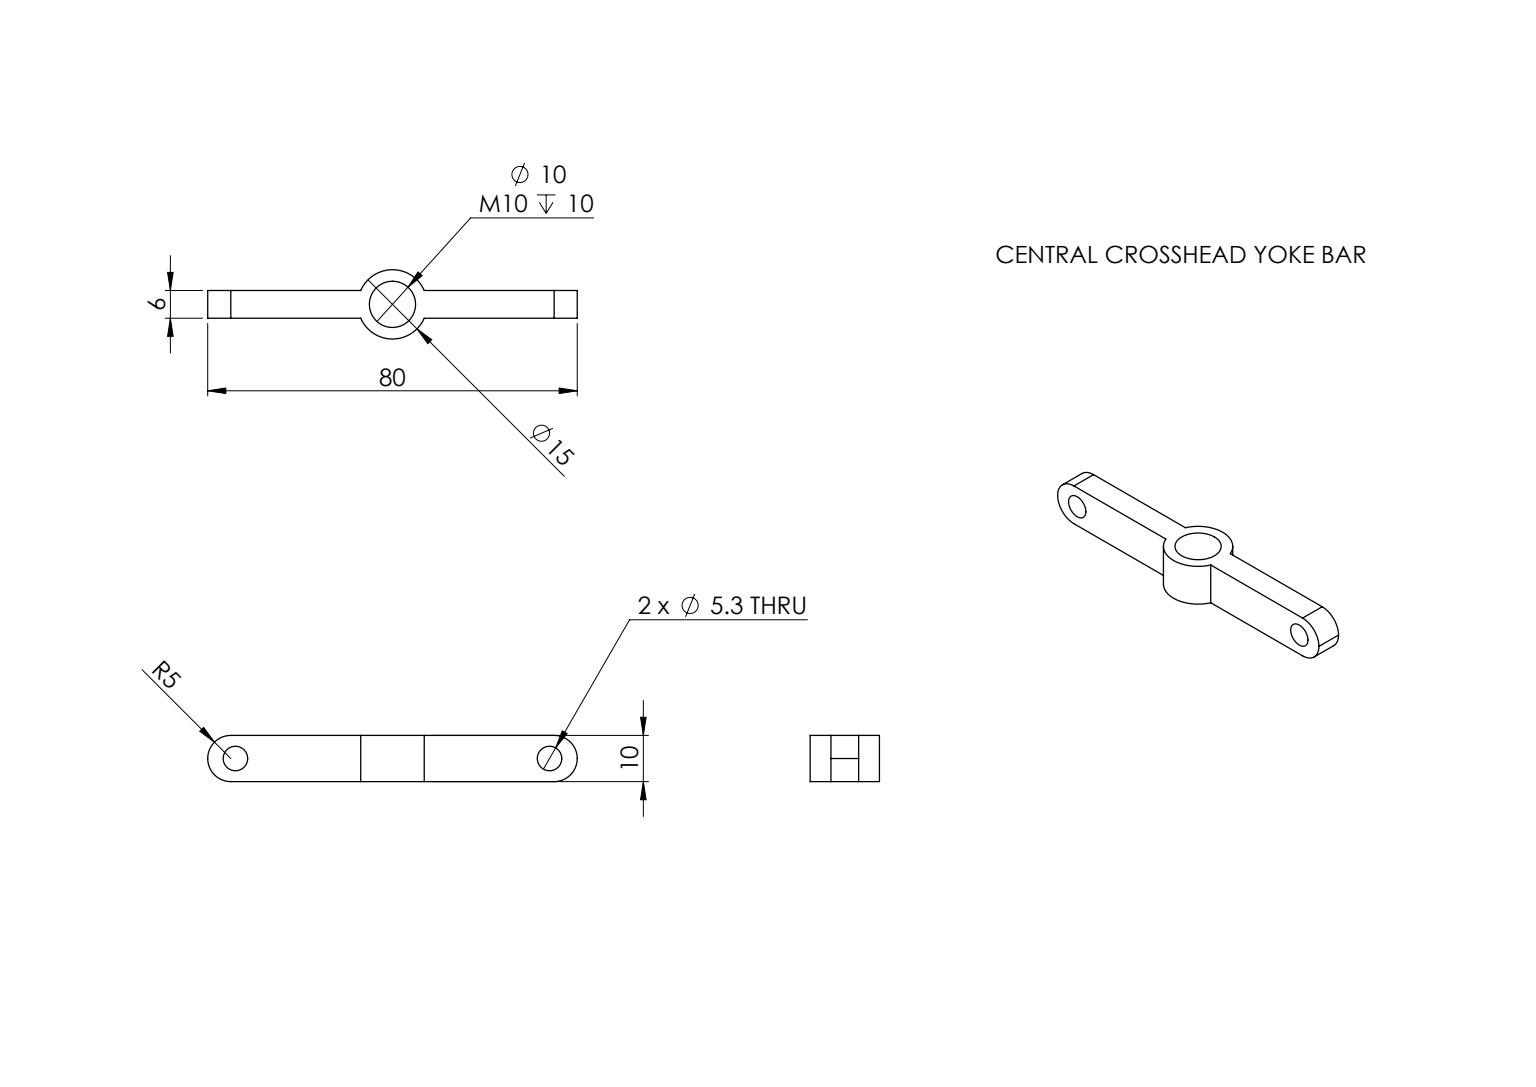
ISO-10303-21;
HEADER;
FILE_DESCRIPTION (('STEP AP214'),
    '1' );
FILE_NAME ('Central Crosshead Yoke Bar.step',
    '2026-10-22T13:24:12',
    ( '' ),
    ( '' ),
    'SwSTEP 2.0',
    'SolidWorks 2026',
    '' );
FILE_SCHEMA (( 'AUTOMOTIVE_DESIGN' ));
ENDSEC;

DATA;
#8=ORIENTED_EDGE ( 'NONE', *, *, #1854, .F. ) ;
#23=VERTEX_POINT ( 'NONE', #2540 ) ;
#29=ORIENTED_EDGE ( 'NONE', *, *, #1848, .F. ) ;
#30=DIRECTION ( 'NONE',  ( -1.000000000000000000, 0.000000000000000000, 0.000000000000000000 ) ) ;
#34=ORIENTED_EDGE ( 'NONE', *, *, #947, .F. ) ;
#40=SURFACE_SIDE_STYLE ('',( #2060 ) ) ;
#41=ORIENTED_EDGE ( 'NONE', *, *, #2625, .F. ) ;
#43=DIRECTION ( 'NONE',  ( -0.000000000000000000, -1.000000000000000000, -0.000000000000000000 ) ) ;
#44=DIRECTION ( 'NONE',  ( 0.000000000000000000, 1.000000000000000000, 0.000000000000000000 ) ) ;
#48=CARTESIAN_POINT ( 'NONE',  ( -34.99999999999999289, -20.00000000000000000, 3.000000000000000000 ) ) ;
#49=CIRCLE ( 'NONE', #831, 7.500000000000000888 ) ;
#50=FACE_BOUND ( 'NONE', #2831, .T. ) ;
#61=DIRECTION ( 'NONE',  ( 1.000000000000000000, 0.000000000000000000, 0.000000000000000000 ) ) ;
#64=ORIENTED_EDGE ( 'NONE', *, *, #1925, .F. ) ;
#65=EDGE_CURVE ( 'NONE', #415, #110, #2593, .T. ) ;
#67=AXIS2_PLACEMENT_3D ( 'NONE', #278, #535, #1657 ) ;
#80=EDGE_CURVE ( 'NONE', #1900, #237, #994, .T. ) ;
#84=CARTESIAN_POINT ( 'NONE',  ( -39.99999999999999289, -30.00000000000000000, -3.000000000000000000 ) ) ;
#97=STYLED_ITEM('',(#2949),#2534);
#99=CARTESIAN_POINT ( 'NONE',  ( -31.35000000000001563, -25.00000000000000000, -3.000000000000001332 ) ) ;
#100=EDGE_LOOP ( 'NONE', ( #2045, #2281 ) ) ;
#101=MECHANICAL_DESIGN_GEOMETRIC_PRESENTATION_REPRESENTATION('',(#833),#2032);
#102=DIRECTION ( 'NONE',  ( -1.000000000000000000, 0.000000000000000000, 0.000000000000000000 ) ) ;
#110=VERTEX_POINT ( 'NONE', #332 ) ;
#112=VECTOR ( 'NONE', #2880, 1000.000000000000000 ) ;
#115=EDGE_LOOP ( 'NONE', ( #29, #1418, #842, #2140 ) ) ;
#130=ORIENTED_EDGE ( 'NONE', *, *, #1665, .T. ) ;
#133=DIRECTION ( 'NONE',  ( -2.312964634635742661E-15, 0.000000000000000000, -1.000000000000000000 ) ) ;
#135=ORIENTED_EDGE ( 'NONE', *, *, #1188, .F. ) ;
#144=DIRECTION ( 'NONE',  ( 1.000000000000000000, 0.000000000000000000, -2.341876692568690761E-15 ) ) ;
#147=CYLINDRICAL_SURFACE ( 'NONE', #663, 5.000000000000000888 ) ;
#157=EDGE_LOOP ( 'NONE', ( #1667, #2865, #926, #590, #162 ) ) ;
#158=VECTOR ( 'NONE', #1568, 1000.000000000000000 ) ;
#162=ORIENTED_EDGE ( 'NONE', *, *, #1048, .T. ) ;
#163=FACE_OUTER_BOUND ( 'NONE', #394, .T. ) ;
#165=EDGE_LOOP ( 'NONE', ( #896, #1637 ) ) ;
#166=( NAMED_UNIT ( * ) SI_UNIT ( $, .STERADIAN. ) SOLID_ANGLE_UNIT ( ) );
#170=CARTESIAN_POINT ( 'NONE',  ( 34.00000000000000000, -25.00000000000000000, -3.000000000000001332 ) ) ;
#174=ORIENTED_EDGE ( 'NONE', *, *, #892, .F. ) ;
#179=CARTESIAN_POINT ( 'NONE',  ( -6.873863542433761076, -20.00000000000000000, 3.000000000000000000 ) ) ;
#187=DIRECTION ( 'NONE',  ( -0.000000000000000000, -1.000000000000000000, -0.000000000000000000 ) ) ;
#193=AXIS2_PLACEMENT_3D ( 'NONE', #1698, #1267, #144 ) ;
#200=FACE_OUTER_BOUND ( 'NONE', #1652, .T. ) ;
#203=ORIENTED_EDGE ( 'NONE', *, *, #1188, .T. ) ;
#206=AXIS2_PLACEMENT_3D ( 'NONE', #1277, #1543, #609 ) ;
#209=DIRECTION ( 'NONE',  ( 0.000000000000000000, 0.000000000000000000, 1.000000000000000000 ) ) ;
#218=VERTEX_POINT ( 'NONE', #1654 ) ;
#220=PLANE ( 'NONE',  #1032 ) ;
#221=DIRECTION ( 'NONE',  ( 0.000000000000000000, 0.000000000000000000, -1.000000000000000000 ) ) ;
#227=CARTESIAN_POINT ( 'NONE',  ( 0.000000000000000000, -30.00000000000000000, 0.000000000000000000 ) ) ;
#228=DIRECTION ( 'NONE',  ( -0.000000000000000000, -1.000000000000000000, -0.000000000000000000 ) ) ;
#231=CARTESIAN_POINT ( 'NONE',  ( 0.000000000000000000, 0.000000000000000000, 0.000000000000000000 ) ) ;
#237=VERTEX_POINT ( 'NONE', #1323 ) ;
#239=AXIS2_PLACEMENT_3D ( 'NONE', #267, #1061, #1149 ) ;
#241=ORIENTED_EDGE ( 'NONE', *, *, #2815, .T. ) ;
#244=ADVANCED_FACE ( 'NONE', ( #397 ), #1289, .T. ) ;
#246=EDGE_CURVE ( 'NONE', #218, #2864, #2203, .T. ) ;
#256=VECTOR ( 'NONE', #2846, 1000.000000000000000 ) ;
#258=EDGE_LOOP ( 'NONE', ( #2402, #1202, #483, #1037 ) ) ;
#259=LINE ( 'NONE', #2309, #1324 ) ;
#264=EDGE_LOOP ( 'NONE', ( #1087, #283, #1551, #1453 ) ) ;
#267=CARTESIAN_POINT ( 'NONE',  ( -34.00000000000000000, -25.00000000000000000, -3.000000000000000000 ) ) ;
#271=ADVANCED_FACE ( 'NONE', ( #1528 ), #592, .T. ) ;
#275=ORIENTED_EDGE ( 'NONE', *, *, #574, .T. ) ;
#276=DIRECTION ( 'NONE',  ( -1.000000000000000000, 0.000000000000000000, 0.000000000000000000 ) ) ;
#278=CARTESIAN_POINT ( 'NONE',  ( 34.00000000000000000, -25.00000000000000000, -3.000000000000001332 ) ) ;
#283=ORIENTED_EDGE ( 'NONE', *, *, #2016, .F. ) ;
#284=DIRECTION ( 'NONE',  ( 0.000000000000000000, -0.000000000000000000, 1.000000000000000000 ) ) ;
#285=( GEOMETRIC_REPRESENTATION_CONTEXT ( 3 ) GLOBAL_UNCERTAINTY_ASSIGNED_CONTEXT ( ( #2051 ) ) GLOBAL_UNIT_ASSIGNED_CONTEXT ( ( #2879, #1600, #166 ) ) REPRESENTATION_CONTEXT ( 'NONE', 'WORKASPACE' ) );
#292=LINE ( 'NONE', #1175, #703 ) ;
#293=EDGE_CURVE ( 'NONE', #444, #937, #848, .T. ) ;
#297=CARTESIAN_POINT ( 'NONE',  ( 36.64999999999999147, -25.00000000000000000, -3.000000000000001332 ) ) ;
#299=AXIS2_PLACEMENT_3D ( 'NONE', #2890, #509, #2101 ) ;
#304=ORIENTED_EDGE ( 'NONE', *, *, #2625, .T. ) ;
#313=CARTESIAN_POINT ( 'NONE',  ( 0.000000000000000000, -30.00000000000000000, 0.000000000000000000 ) ) ;
#314=ORIENTED_EDGE ( 'NONE', *, *, #2815, .F. ) ;
#318=ADVANCED_FACE ( 'NONE', ( #200 ), #1081, .F. ) ;
#320=ORIENTED_EDGE ( 'NONE', *, *, #2703, .T. ) ;
#323=DIRECTION ( 'NONE',  ( 0.000000000000000000, 1.000000000000000000, 0.000000000000000000 ) ) ;
#327=VERTEX_POINT ( 'NONE', #425 ) ;
#328=CIRCLE ( 'NONE', #2312, 7.500000000000000888 ) ;
#331=CIRCLE ( 'NONE', #981, 5.000000000000000888 ) ;
#332=CARTESIAN_POINT ( 'NONE',  ( 6.873863542433761076, -30.00000000000000000, 3.000000000000000000 ) ) ;
#335=CARTESIAN_POINT ( 'NONE',  ( -34.00000000000000000, -25.00000000000000000, -3.000000000000001332 ) ) ;
#343=AXIS2_PLACEMENT_3D ( 'NONE', #865, #2176, #2444 ) ;
#345=CARTESIAN_POINT ( 'NONE',  ( 6.873863542433761076, -30.00000000000000000, 3.000000000000000000 ) ) ;
#348=VECTOR ( 'NONE', #1776, 1000.000000000000000 ) ;
#354=CARTESIAN_POINT ( 'NONE',  ( 0.000000000000000000, -30.00000000000000000, 0.000000000000000000 ) ) ;
#362=CARTESIAN_POINT ( 'NONE',  ( -34.00000000000000000, -25.00000000000000000, -3.000000000000001332 ) ) ;
#367=DIRECTION ( 'NONE',  ( -0.000000000000000000, -0.000000000000000000, -1.000000000000000000 ) ) ;
#368=ORIENTED_EDGE ( 'NONE', *, *, #2549, .T. ) ;
#370=ADVANCED_FACE ( 'NONE', ( #2055, #484 ), #680, .T. ) ;
#377=CIRCLE ( 'NONE', #602, 7.500000000000000888 ) ;
#383=CIRCLE ( 'NONE', #2037, 2.649999999999992806 ) ;
#393=DIRECTION ( 'NONE',  ( -0.000000000000000000, -0.000000000000000000, -1.000000000000000000 ) ) ;
#394=EDGE_LOOP ( 'NONE', ( #2893, #2844, #823, #135 ) ) ;
#395=CYLINDRICAL_SURFACE ( 'NONE', #239, 2.649999999999992806 ) ;
#397=FACE_OUTER_BOUND ( 'NONE', #2041, .T. ) ;
#403=CARTESIAN_POINT ( 'NONE',  ( -31.35000000000000853, -25.00000000000000000, -3.000000000000000000 ) ) ;
#407=ORIENTED_EDGE ( 'NONE', *, *, #246, .F. ) ;
#411=ORIENTED_EDGE ( 'NONE', *, *, #1925, .T. ) ;
#415=VERTEX_POINT ( 'NONE', #2763 ) ;
#425=CARTESIAN_POINT ( 'NONE',  ( 40.00000000000002132, -24.99999999999999645, 3.000000000000000000 ) ) ;
#426=ADVANCED_FACE ( 'NONE', ( #1140 ), #715, .F. ) ;
#429=ORIENTED_EDGE ( 'NONE', *, *, #1791, .T. ) ;
#442=ORIENTED_EDGE ( 'NONE', *, *, #787, .T. ) ;
#443=CARTESIAN_POINT ( 'NONE',  ( -34.99999999999999289, -30.00000000000000000, -3.000000000000000000 ) ) ;
#444=VERTEX_POINT ( 'NONE', #48 ) ;
#448=LINE ( 'NONE', #1584, #348 ) ;
#449=ADVANCED_FACE ( 'NONE', ( #1389 ), #497, .T. ) ;
#450=ORIENTED_EDGE ( 'NONE', *, *, #895, .F. ) ;
#451=CARTESIAN_POINT ( 'NONE',  ( -39.99999999999999289, -30.00000000000000000, -3.000000000000000000 ) ) ;
#458=CARTESIAN_POINT ( 'NONE',  ( 0.000000000000000000, -30.00000000000000000, 7.500000000000000888 ) ) ;
#461=AXIS2_PLACEMENT_3D ( 'NONE', #84, #2266, #924 ) ;
#464=CARTESIAN_POINT ( 'NONE',  ( -36.64999999999999858, -25.00000000000000000, 3.000000000000000000 ) ) ;
#465=( GEOMETRIC_REPRESENTATION_CONTEXT ( 3 ) GLOBAL_UNCERTAINTY_ASSIGNED_CONTEXT ( ( #646 ) ) GLOBAL_UNIT_ASSIGNED_CONTEXT ( ( #1799, #1594, #1071 ) ) REPRESENTATION_CONTEXT ( 'NONE', 'WORKASPACE' ) );
#468=CARTESIAN_POINT ( 'NONE',  ( 34.00000000000000000, -25.00000000000000000, -3.000000000000000000 ) ) ;
#474=PRESENTATION_STYLE_ASSIGNMENT (( #1827 ) ) ;
#475=AXIS2_PLACEMENT_3D ( 'NONE', #2390, #2583, #2376 ) ;
#476=VERTEX_POINT ( 'NONE', #669 ) ;
#483=ORIENTED_EDGE ( 'NONE', *, *, #1201, .T. ) ;
#484=FACE_OUTER_BOUND ( 'NONE', #157, .T. ) ;
#490=EDGE_CURVE ( 'NONE', #237, #444, #259, .T. ) ;
#492=DIRECTION ( 'NONE',  ( 0.000000000000000000, 0.000000000000000000, -1.000000000000000000 ) ) ;
#497=CYLINDRICAL_SURFACE ( 'NONE', #2520, 7.500000000000000888 ) ;
#498=CARTESIAN_POINT ( 'NONE',  ( 0.000000000000000000, -30.00000000000000000, 0.000000000000000000 ) ) ;
#504=FACE_OUTER_BOUND ( 'NONE', #726, .T. ) ;
#509=DIRECTION ( 'NONE',  ( -0.000000000000000000, -1.000000000000000000, -0.000000000000000000 ) ) ;
#512=CIRCLE ( 'NONE', #889, 5.000000000000000000 ) ;
#520=DIRECTION ( 'NONE',  ( -1.000000000000000000, -0.000000000000000000, -0.000000000000000000 ) ) ;
#525=VECTOR ( 'NONE', #1246, 1000.000000000000000 ) ;
#526=AXIS2_PLACEMENT_3D ( 'NONE', #2675, #2659, #1946 ) ;
#528=CIRCLE ( 'NONE', #1435, 7.500000000000000888 ) ;
#529=DIRECTION ( 'NONE',  ( 0.000000000000000000, 1.000000000000000000, 0.000000000000000000 ) ) ;
#532=EDGE_CURVE ( 'NONE', #2405, #2811, #1844, .T. ) ;
#533=CARTESIAN_POINT ( 'NONE',  ( 0.000000000000000000, -20.00000000000000000, 0.000000000000000000 ) ) ;
#535=DIRECTION ( 'NONE',  ( -0.000000000000000000, -0.000000000000000000, -1.000000000000000000 ) ) ;
#549=ORIENTED_EDGE ( 'NONE', *, *, #293, .F. ) ;
#556=ORIENTED_EDGE ( 'NONE', *, *, #2594, .T. ) ;
#562=ADVANCED_FACE ( 'NONE', ( #163 ), #147, .T. ) ;
#568=DIRECTION ( 'NONE',  ( -1.000000000000000000, -0.000000000000000000, -0.000000000000000000 ) ) ;
#573=DIRECTION ( 'NONE',  ( 2.312964634635742661E-15, -0.000000000000000000, 1.000000000000000000 ) ) ;
#574=EDGE_CURVE ( 'NONE', #218, #2093, #528, .T. ) ;
#590=ORIENTED_EDGE ( 'NONE', *, *, #1935, .F. ) ;
#592=CYLINDRICAL_SURFACE ( 'NONE', #206, 5.000000000000000888 ) ;
#597=EDGE_CURVE ( 'NONE', #476, #1951, #2616, .T. ) ;
#599=VECTOR ( 'NONE', #367, 1000.000000000000000 ) ;
#602=AXIS2_PLACEMENT_3D ( 'NONE', #2789, #44, #1896 ) ;
#609=DIRECTION ( 'NONE',  ( 1.000000000000000000, 0.000000000000000000, 0.000000000000000000 ) ) ;
#618=CARTESIAN_POINT ( 'NONE',  ( 6.873863542433758411, -20.00000000000000000, -3.000000000000000000 ) ) ;
#619=ORIENTED_EDGE ( 'NONE', *, *, #769, .F. ) ;
#630=DIRECTION ( 'NONE',  ( 0.000000000000000000, 1.000000000000000000, 0.000000000000000000 ) ) ;
#640=VERTEX_POINT ( 'NONE', #1919 ) ;
#644=AXIS2_PLACEMENT_3D ( 'NONE', #2442, #863, #2458 ) ;
#646=UNCERTAINTY_MEASURE_WITH_UNIT (LENGTH_MEASURE( 1.000000000000000082E-05 ), #1799, 'distance_accuracy_value', 'NONE');
#648=CIRCLE ( 'NONE', #1973, 2.649999999999992806 ) ;
#650=AXIS2_PLACEMENT_3D ( 'NONE', #975, #1444, #1863 ) ;
#651=EDGE_CURVE ( 'NONE', #2441, #2627, #2183, .T. ) ;
#655=CARTESIAN_POINT ( 'NONE',  ( 0.000000000000000000, -30.00000000000000000, 0.000000000000000000 ) ) ;
#658=CARTESIAN_POINT ( 'NONE',  ( 0.000000000000000000, -20.00000000000000000, 0.000000000000000000 ) ) ;
#661=EDGE_LOOP ( 'NONE', ( #2878, #368, #429, #1847, #2459 ) ) ;
#662=LINE ( 'NONE', #403, #158 ) ;
#663=AXIS2_PLACEMENT_3D ( 'NONE', #1469, #133, #1035 ) ;
#666=CARTESIAN_POINT ( 'NONE',  ( 40.00000000000000711, -24.99999999999999645, -3.000000000000000000 ) ) ;
#668=ORIENTED_EDGE ( 'NONE', *, *, #651, .F. ) ;
#669=CARTESIAN_POINT ( 'NONE',  ( -36.64999999999999147, -25.00000000000000000, -3.000000000000001332 ) ) ;
#677=ORIENTED_EDGE ( 'NONE', *, *, #2343, .T. ) ;
#680=PLANE ( 'NONE',  #2378 ) ;
#692=CYLINDRICAL_SURFACE ( 'NONE', #2848, 2.649999999999992806 ) ;
#703=VECTOR ( 'NONE', #1826, 1000.000000000000000 ) ;
#713=CIRCLE ( 'NONE', #807, 2.649999999999985700 ) ;
#715=CYLINDRICAL_SURFACE ( 'NONE', #1894, 2.649999999999992806 ) ;
#718=EDGE_LOOP ( 'NONE', ( #2082, #993, #8, #549 ) ) ;
#726=EDGE_LOOP ( 'NONE', ( #2547, #2181, #1068, #1158, #556 ) ) ;
#733=CARTESIAN_POINT ( 'NONE',  ( -34.99999999999999289, -24.99999999999999645, -3.000000000000000000 ) ) ;
#738=EDGE_CURVE ( 'NONE', #1558, #23, #1382, .T. ) ;
#753=DIRECTION ( 'NONE',  ( -0.000000000000000000, -1.000000000000000000, -0.000000000000000000 ) ) ;
#765=CARTESIAN_POINT ( 'NONE',  ( -34.99999999999999289, -24.99999999999999645, 3.000000000000000000 ) ) ;
#769=EDGE_CURVE ( 'NONE', #2627, #2492, #859, .T. ) ;
#772=VERTEX_POINT ( 'NONE', #2471 ) ;
#778=( LENGTH_UNIT ( ) NAMED_UNIT ( * ) SI_UNIT ( .MILLI., .METRE. ) );
#787=EDGE_CURVE ( 'NONE', #2799, #1951, #662, .T. ) ;
#796=EDGE_CURVE ( 'NONE', #444, #2492, #1743, .T. ) ;
#807=AXIS2_PLACEMENT_3D ( 'NONE', #335, #2364, #102 ) ;
#815=EDGE_CURVE ( 'NONE', #2093, #1704, #1830, .T. ) ;
#822=DIRECTION ( 'NONE',  ( 1.000000000000000000, 0.000000000000000000, 0.000000000000000000 ) ) ;
#823=ORIENTED_EDGE ( 'NONE', *, *, #2549, .F. ) ;
#825=EDGE_CURVE ( 'NONE', #937, #2441, #905, .T. ) ;
#826=ORIENTED_EDGE ( 'NONE', *, *, #738, .T. ) ;
#831=AXIS2_PLACEMENT_3D ( 'NONE', #1245, #529, #1690 ) ;
#833=STYLED_ITEM ( 'NONE', ( #474 ), #1110 ) ;
#838=CIRCLE ( 'NONE', #1074, 2.649999999999992806 ) ;
#839=CARTESIAN_POINT ( 'NONE',  ( -39.99999999999999289, -20.00000000000000000, 3.000000000000000000 ) ) ;
#840=AXIS2_PLACEMENT_3D ( 'NONE', #1949, #2873, #2632 ) ;
#842=ORIENTED_EDGE ( 'NONE', *, *, #2826, .F. ) ;
#848=CIRCLE ( 'NONE', #526, 5.000000000000000888 ) ;
#852=EDGE_CURVE ( 'NONE', #1704, #1900, #1232, .T. ) ;
#859=LINE ( 'NONE', #2697, #2233 ) ;
#861=CARTESIAN_POINT ( 'NONE',  ( 35.00000000000001421, -20.00000000000000000, -8.095376221225103140E-14 ) ) ;
#863=DIRECTION ( 'NONE',  ( -0.000000000000000000, -1.000000000000000000, -0.000000000000000000 ) ) ;
#865=CARTESIAN_POINT ( 'NONE',  ( 0.000000000000000000, -30.00000000000000000, 0.000000000000000000 ) ) ;
#868=ORIENTED_EDGE ( 'NONE', *, *, #796, .F. ) ;
#871=ORIENTED_EDGE ( 'NONE', *, *, #2130, .T. ) ;
#875=LINE ( 'NONE', #1571, #1613 ) ;
#881=EDGE_CURVE ( 'NONE', #327, #1027, #1663, .T. ) ;
#884=ORIENTED_EDGE ( 'NONE', *, *, #815, .F. ) ;
#889=AXIS2_PLACEMENT_3D ( 'NONE', #2003, #187, #221 ) ;
#891=DIRECTION ( 'NONE',  ( -2.312964634635742661E-15, 0.000000000000000000, -1.000000000000000000 ) ) ;
#892=EDGE_CURVE ( 'NONE', #1101, #476, #2304, .T. ) ;
#895=EDGE_CURVE ( 'NONE', #772, #2668, #1610, .T. ) ;
#896=ORIENTED_EDGE ( 'NONE', *, *, #597, .F. ) ;
#897=DIRECTION ( 'NONE',  ( -1.000000000000000000, 0.000000000000000000, -0.000000000000000000 ) ) ;
#899=CARTESIAN_POINT ( 'NONE',  ( -6.873863542433758411, -30.00000000000000000, -3.000000000000000000 ) ) ;
#901=CARTESIAN_POINT ( 'NONE',  ( -34.00000000000000000, -25.00000000000000000, 3.000000000000000000 ) ) ;
#905=CIRCLE ( 'NONE', #2573, 5.000000000000000888 ) ;
#922=DIRECTION ( 'NONE',  ( 0.000000000000000000, 1.000000000000000000, 0.000000000000000000 ) ) ;
#924=DIRECTION ( 'NONE',  ( -1.000000000000000000, 0.000000000000000000, -0.000000000000000000 ) ) ;
#926=ORIENTED_EDGE ( 'NONE', *, *, #80, .T. ) ;
#929=EDGE_LOOP ( 'NONE', ( #2115, #2050, #1166, #1699 ) ) ;
#935=CYLINDRICAL_SURFACE ( 'NONE', #1220, 5.000000000000000000 ) ;
#937=VERTEX_POINT ( 'NONE', #974 ) ;
#940=FACE_OUTER_BOUND ( 'NONE', #1400, .T. ) ;
#947=EDGE_CURVE ( 'NONE', #23, #2668, #2739, .T. ) ;
#951=DIRECTION ( 'NONE',  ( 0.000000000000000000, 0.000000000000000000, -1.000000000000000000 ) ) ;
#952=AXIS2_PLACEMENT_3D ( 'NONE', #733, #492, #30 ) ;
#974=CARTESIAN_POINT ( 'NONE',  ( -39.99999999999999289, -25.00000000000000000, 3.000000000000000000 ) ) ;
#975=CARTESIAN_POINT ( 'NONE',  ( -39.99999999999999289, -30.00000000000000000, 3.000000000000000000 ) ) ;
#981=AXIS2_PLACEMENT_3D ( 'NONE', #1993, #2687, #1512 ) ;
#989=ORIENTED_EDGE ( 'NONE', *, *, #2428, .F. ) ;
#993=ORIENTED_EDGE ( 'NONE', *, *, #80, .F. ) ;
#994=CIRCLE ( 'NONE', #475, 4.999999999999997335 ) ;
#998=VERTEX_POINT ( 'NONE', #1862 ) ;
#999=CYLINDRICAL_SURFACE ( 'NONE', #2840, 7.500000000000000888 ) ;
#1000=EDGE_CURVE ( 'NONE', #1951, #476, #713, .T. ) ;
#1003=ORIENTED_EDGE ( 'NONE', *, *, #651, .T. ) ;
#1008=EDGE_LOOP ( 'NONE', ( #1801, #1380, #1747, #1345 ) ) ;
#1022=VECTOR ( 'NONE', #1645, 1000.000000000000000 ) ;
#1026=DIRECTION ( 'NONE',  ( 0.000000000000000000, -0.000000000000000000, -1.000000000000000000 ) ) ;
#1027=VERTEX_POINT ( 'NONE', #2488 ) ;
#1029=VECTOR ( 'NONE', #2352, 1000.000000000000000 ) ;
#1031=CYLINDRICAL_SURFACE ( 'NONE', #193, 4.999999999999997335 ) ;
#1032=AXIS2_PLACEMENT_3D ( 'NONE', #658, #630, #2207 ) ;
#1035=DIRECTION ( 'NONE',  ( -1.000000000000000000, 0.000000000000000000, 2.312964634635741478E-15 ) ) ;
#1037=ORIENTED_EDGE ( 'NONE', *, *, #2918, .T. ) ;
#1041=DIRECTION ( 'NONE',  ( -1.000000000000000000, 0.000000000000000000, 0.000000000000000000 ) ) ;
#1043=VERTEX_POINT ( 'NONE', #666 ) ;
#1044=FACE_OUTER_BOUND ( 'NONE', #1542, .T. ) ;
#1046=ORIENTED_EDGE ( 'NONE', *, *, #490, .T. ) ;
#1048=EDGE_CURVE ( 'NONE', #2373, #2093, #448, .T. ) ;
#1059=DIRECTION ( 'NONE',  ( 0.000000000000000000, 0.000000000000000000, 1.000000000000000000 ) ) ;
#1061=DIRECTION ( 'NONE',  ( -0.000000000000000000, -0.000000000000000000, -1.000000000000000000 ) ) ;
#1064=VECTOR ( 'NONE', #568, 1000.000000000000000 ) ;
#1068=ORIENTED_EDGE ( 'NONE', *, *, #1521, .F. ) ;
#1071=( NAMED_UNIT ( * ) SI_UNIT ( $, .STERADIAN. ) SOLID_ANGLE_UNIT ( ) );
#1074=AXIS2_PLACEMENT_3D ( 'NONE', #2545, #1446, #61 ) ;
#1075=DIRECTION ( 'NONE',  ( 1.000000000000000000, 0.000000000000000000, 0.000000000000000000 ) ) ;
#1076=FACE_BOUND ( 'NONE', #2478, .T. ) ;
#1081=CYLINDRICAL_SURFACE ( 'NONE', #2136, 2.649999999999992806 ) ;
#1087=ORIENTED_EDGE ( 'NONE', *, *, #852, .F. ) ;
#1097=EDGE_CURVE ( 'NONE', #998, #218, #875, .T. ) ;
#1101=VERTEX_POINT ( 'NONE', #464 ) ;
#1107=PRODUCT_DEFINITION ( 'UNKNOWN', '', #1218, #2292 ) ;
#1110=ADVANCED_BREP_SHAPE_REPRESENTATION ( '', ( #2534, #2652 ), #465 ) ;
#1140=FACE_OUTER_BOUND ( 'NONE', #2387, .T. ) ;
#1145=FILL_AREA_STYLE_COLOUR ( '', #2125 ) ;
#1147=CARTESIAN_POINT ( 'NONE',  ( -34.99999999999999289, -24.99999999999999645, 3.000000000000000000 ) ) ;
#1149=DIRECTION ( 'NONE',  ( -1.000000000000000000, 0.000000000000000000, 0.000000000000000000 ) ) ;
#1150=DIRECTION ( 'NONE',  ( -0.000000000000000000, -1.000000000000000000, -0.000000000000000000 ) ) ;
#1153=DIRECTION ( 'NONE',  ( 0.000000000000000000, 1.000000000000000000, 0.000000000000000000 ) ) ;
#1158=ORIENTED_EDGE ( 'NONE', *, *, #65, .T. ) ;
#1159=DIRECTION ( 'NONE',  ( 1.000000000000000000, 0.000000000000000000, 0.000000000000000000 ) ) ;
#1166=ORIENTED_EDGE ( 'NONE', *, *, #2153, .T. ) ;
#1175=CARTESIAN_POINT ( 'NONE',  ( 40.00000000000000711, -24.99999999999999645, -3.000000000000000888 ) ) ;
#1181=CARTESIAN_POINT ( 'NONE',  ( -39.99999999999999289, -30.00000000000000000, 3.000000000000000000 ) ) ;
#1183=VECTOR ( 'NONE', #2772, 1000.000000000000000 ) ;
#1184=PRODUCT_DEFINITION_SHAPE ( 'NONE', 'NONE',  #1107 ) ;
#1188=EDGE_CURVE ( 'NONE', #1027, #2297, #1989, .T. ) ;
#1196=CARTESIAN_POINT ( 'NONE',  ( 35.00000000000002132, -25.00000000000000000, 3.000000000000000000 ) ) ;
#1201=EDGE_CURVE ( 'NONE', #2405, #1292, #2578, .T. ) ;
#1202=ORIENTED_EDGE ( 'NONE', *, *, #532, .F. ) ;
#1203=FACE_OUTER_BOUND ( 'NONE', #1737, .T. ) ;
#1208=DIRECTION ( 'NONE',  ( 0.000000000000000000, 0.000000000000000000, 1.000000000000000000 ) ) ;
#1211=ORIENTED_EDGE ( 'NONE', *, *, #1935, .T. ) ;
#1214=ADVANCED_FACE ( 'NONE', ( #1881 ), #692, .F. ) ;
#1215=ORIENTED_EDGE ( 'NONE', *, *, #947, .T. ) ;
#1218=PRODUCT_DEFINITION_FORMATION_WITH_SPECIFIED_SOURCE ( 'ANY', '', #2791, .NOT_KNOWN. ) ;
#1219=EDGE_LOOP ( 'NONE', ( #1459, #203, #871, #411, #1211, #1046, #2542, #1438, #320 ) ) ;
#1220=AXIS2_PLACEMENT_3D ( 'NONE', #313, #753, #951 ) ;
#1227=CARTESIAN_POINT ( 'NONE',  ( -31.35000000000000853, -25.00000000000000000, 3.000000000000000000 ) ) ;
#1231=( NAMED_UNIT ( * ) SI_UNIT ( $, .STERADIAN. ) SOLID_ANGLE_UNIT ( ) );
#1232=CIRCLE ( 'NONE', #952, 4.999999999999997335 ) ;
#1240=FACE_BOUND ( 'NONE', #2054, .T. ) ;
#1243=CARTESIAN_POINT ( 'NONE',  ( 0.000000000000000000, -30.00000000000000000, 0.000000000000000000 ) ) ;
#1245=CARTESIAN_POINT ( 'NONE',  ( 0.000000000000000000, -20.00000000000000000, 0.000000000000000000 ) ) ;
#1246=DIRECTION ( 'NONE',  ( -0.000000000000000000, -1.000000000000000000, -0.000000000000000000 ) ) ;
#1250=PLANE ( 'NONE',  #1268 ) ;
#1257=CARTESIAN_POINT ( 'NONE',  ( -6.873863542433761076, -20.00000000000000000, -3.000000000000000000 ) ) ;
#1264=EDGE_CURVE ( 'NONE', #2799, #1101, #838, .T. ) ;
#1267=DIRECTION ( 'NONE',  ( 2.312964634635742661E-15, -0.000000000000000000, 1.000000000000000000 ) ) ;
#1268=AXIS2_PLACEMENT_3D ( 'NONE', #2195, #2149, #2165 ) ;
#1277=CARTESIAN_POINT ( 'NONE',  ( -34.99999999999999289, -25.00000000000000000, 0.000000000000000000 ) ) ;
#1289=CYLINDRICAL_SURFACE ( 'NONE', #343, 7.500000000000000888 ) ;
#1292=VERTEX_POINT ( 'NONE', #2341 ) ;
#1295=DIRECTION ( 'NONE',  ( 1.000000000000000000, 0.000000000000000000, 0.000000000000000000 ) ) ;
#1299=ADVANCED_FACE ( 'NONE', ( #2099 ), #935, .F. ) ;
#1302=VECTOR ( 'NONE', #2012, 1000.000000000000000 ) ;
#1309=DIRECTION ( 'NONE',  ( 1.000000000000000000, 0.000000000000000000, 0.000000000000000000 ) ) ;
#1312=ORIENTED_EDGE ( 'NONE', *, *, #1763, .T. ) ;
#1318=DIRECTION ( 'NONE',  ( -1.000000000000000000, -0.000000000000000000, -0.000000000000000000 ) ) ;
#1322=ORIENTED_EDGE ( 'NONE', *, *, #895, .T. ) ;
#1323=CARTESIAN_POINT ( 'NONE',  ( -34.99999999999999289, -20.00000000000000000, -3.000000000000000000 ) ) ;
#1324=VECTOR ( 'NONE', #284, 1000.000000000000000 ) ;
#1327=AXIS2_PLACEMENT_3D ( 'NONE', #362, #393, #2876 ) ;
#1334=UNCERTAINTY_MEASURE_WITH_UNIT (LENGTH_MEASURE( 1.000000000000000082E-05 ), #778, 'distance_accuracy_value', 'NONE');
#1345=ORIENTED_EDGE ( 'NONE', *, *, #597, .T. ) ;
#1346=DIRECTION ( 'NONE',  ( 0.000000000000000000, 1.000000000000000000, 0.000000000000000000 ) ) ;
#1374=FACE_BOUND ( 'NONE', #2738, .T. ) ;
#1378=DIRECTION ( 'NONE',  ( -0.000000000000000000, -0.000000000000000000, -1.000000000000000000 ) ) ;
#1380=ORIENTED_EDGE ( 'NONE', *, *, #1264, .T. ) ;
#1382=CIRCLE ( 'NONE', #2285, 2.649999999999992806 ) ;
#1385=DIRECTION ( 'NONE',  ( -1.000000000000000000, 0.000000000000000000, 0.000000000000000000 ) ) ;
#1389=FACE_OUTER_BOUND ( 'NONE', #1964, .T. ) ;
#1390=PLANE ( 'NONE',  #1877 ) ;
#1393=LINE ( 'NONE', #2091, #2356 ) ;
#1400=EDGE_LOOP ( 'NONE', ( #1777, #1476, #1991, #2897, #2582, #668, #1757, #884, #2384 ) ) ;
#1401=DIRECTION ( 'NONE',  ( 0.000000000000000000, 0.000000000000000000, 1.000000000000000000 ) ) ;
#1404=ORIENTED_EDGE ( 'NONE', *, *, #1000, .T. ) ;
#1410=LINE ( 'NONE', #2788, #1504 ) ;
#1418=ORIENTED_EDGE ( 'NONE', *, *, #1615, .F. ) ;
#1434=DIRECTION ( 'NONE',  ( -0.000000000000000000, -0.000000000000000000, -1.000000000000000000 ) ) ;
#1435=AXIS2_PLACEMENT_3D ( 'NONE', #1243, #2795, #1059 ) ;
#1438=ORIENTED_EDGE ( 'NONE', *, *, #2428, .T. ) ;
#1440=DIRECTION ( 'NONE',  ( 0.000000000000000000, 1.000000000000000000, 0.000000000000000000 ) ) ;
#1444=DIRECTION ( 'NONE',  ( 0.000000000000000000, 0.000000000000000000, 1.000000000000000000 ) ) ;
#1445=CARTESIAN_POINT ( 'NONE',  ( 0.000000000000000000, -30.00000000000000000, 7.500000000000000888 ) ) ;
#1446=DIRECTION ( 'NONE',  ( 0.000000000000000000, 0.000000000000000000, 1.000000000000000000 ) ) ;
#1453=ORIENTED_EDGE ( 'NONE', *, *, #1854, .T. ) ;
#1456=ADVANCED_FACE ( 'NONE', ( #1076, #504 ), #1660, .T. ) ;
#1458=CIRCLE ( 'NONE', #2596, 2.649999999999985700 ) ;
#1459=ORIENTED_EDGE ( 'NONE', *, *, #1521, .T. ) ;
#1462=VERTEX_POINT ( 'NONE', #2925 ) ;
#1469=CARTESIAN_POINT ( 'NONE',  ( 35.00000000000001421, -25.00000000000000000, -8.095376221225103140E-14 ) ) ;
#1473=FACE_OUTER_BOUND ( 'NONE', #258, .T. ) ;
#1475=LINE ( 'NONE', #1670, #1064 ) ;
#1476=ORIENTED_EDGE ( 'NONE', *, *, #2826, .T. ) ;
#1483=CARTESIAN_POINT ( 'NONE',  ( -34.99999999999999289, -30.00000000000000000, 3.000000000000000000 ) ) ;
#1484=EDGE_CURVE ( 'NONE', #2811, #1462, #1410, .T. ) ;
#1504=VECTOR ( 'NONE', #43, 1000.000000000000000 ) ;
#1506=CYLINDRICAL_SURFACE ( 'NONE', #2896, 4.999999999999997335 ) ;
#1509=CARTESIAN_POINT ( 'NONE',  ( -39.99999999999999289, -30.00000000000000000, 3.000000000000000000 ) ) ;
#1512=DIRECTION ( 'NONE',  ( -1.000000000000000000, 0.000000000000000000, 0.000000000000000000 ) ) ;
#1521=EDGE_CURVE ( 'NONE', #415, #1027, #1851, .T. ) ;
#1528=FACE_OUTER_BOUND ( 'NONE', #718, .T. ) ;
#1542=EDGE_LOOP ( 'NONE', ( #2451, #1576, #1003, #2496, #868 ) ) ;
#1543=DIRECTION ( 'NONE',  ( 0.000000000000000000, -0.000000000000000000, 1.000000000000000000 ) ) ;
#1551=ORIENTED_EDGE ( 'NONE', *, *, #825, .F. ) ;
#1555=CIRCLE ( 'NONE', #840, 4.999999999999997335 ) ;
#1556=VERTEX_POINT ( 'NONE', #1915 ) ;
#1558=VERTEX_POINT ( 'NONE', #2841 ) ;
#1564=ORIENTED_EDGE ( 'NONE', *, *, #2153, .F. ) ;
#1568=DIRECTION ( 'NONE',  ( -0.000000000000000000, -0.000000000000000000, -1.000000000000000000 ) ) ;
#1571=CARTESIAN_POINT ( 'NONE',  ( -39.99999999999999289, -30.00000000000000000, -3.000000000000000000 ) ) ;
#1576=ORIENTED_EDGE ( 'NONE', *, *, #825, .T. ) ;
#1578=ADVANCED_FACE ( 'NONE', ( #1240, #1044 ), #1250, .T. ) ;
#1584=CARTESIAN_POINT ( 'NONE',  ( -6.873863542433761076, -30.00000000000000000, -3.000000000000000000 ) ) ;
#1594=( NAMED_UNIT ( * ) PLANE_ANGLE_UNIT ( ) SI_UNIT ( $, .RADIAN. ) );
#1600=( NAMED_UNIT ( * ) PLANE_ANGLE_UNIT ( ) SI_UNIT ( $, .RADIAN. ) );
#1603=AXIS2_PLACEMENT_3D ( 'NONE', #1984, #2014, #1784 ) ;
#1609=CARTESIAN_POINT ( 'NONE',  ( 35.00000000000000711, -24.99999999999999645, -3.000000000000000444 ) ) ;
#1610=CIRCLE ( 'NONE', #67, 2.649999999999985700 ) ;
#1612=CARTESIAN_POINT ( 'NONE',  ( 36.64999999999999858, -25.00000000000000000, -3.000000000000000000 ) ) ;
#1613=VECTOR ( 'NONE', #1318, 1000.000000000000000 ) ;
#1615=EDGE_CURVE ( 'NONE', #1556, #327, #1555, .T. ) ;
#1618=DIRECTION ( 'NONE',  ( -0.000000000000000000, -0.000000000000000000, -1.000000000000000000 ) ) ;
#1623=ADVANCED_FACE ( 'NONE', ( #1725 ), #1506, .T. ) ;
#1626=ORIENTED_EDGE ( 'NONE', *, *, #2343, .F. ) ;
#1629=LINE ( 'NONE', #1181, #1022 ) ;
#1631=CARTESIAN_POINT ( 'NONE',  ( -34.00000000000000000, -25.00000000000000000, -3.000000000000000000 ) ) ;
#1637=ORIENTED_EDGE ( 'NONE', *, *, #1000, .F. ) ;
#1638=APPLICATION_CONTEXT ( 'automotive_design' ) ;
#1643=CIRCLE ( 'NONE', #1683, 5.000000000000000000 ) ;
#1645=DIRECTION ( 'NONE',  ( 1.000000000000000000, 0.000000000000000000, 0.000000000000000000 ) ) ;
#1652=EDGE_LOOP ( 'NONE', ( #34, #241, #677, #1322 ) ) ;
#1654=CARTESIAN_POINT ( 'NONE',  ( 6.873863542433761076, -30.00000000000000000, -3.000000000000000000 ) ) ;
#1655=DIRECTION ( 'NONE',  ( 0.000000000000000000, 0.000000000000000000, -1.000000000000000000 ) ) ;
#1657=DIRECTION ( 'NONE',  ( -1.000000000000000000, 0.000000000000000000, 0.000000000000000000 ) ) ;
#1660=PLANE ( 'NONE',  #650 ) ;
#1663=CIRCLE ( 'NONE', #1846, 4.999999999999997335 ) ;
#1665=EDGE_CURVE ( 'NONE', #2627, #2914, #2513, .T. ) ;
#1666=DIRECTION ( 'NONE',  ( 0.000000000000000000, 0.000000000000000000, -1.000000000000000000 ) ) ;
#1667=ORIENTED_EDGE ( 'NONE', *, *, #815, .T. ) ;
#1670=CARTESIAN_POINT ( 'NONE',  ( -39.99999999999999289, -20.00000000000000000, -3.000000000000000000 ) ) ;
#1673=DIRECTION ( 'NONE',  ( 0.000000000000000000, 0.000000000000000000, -1.000000000000000000 ) ) ;
#1683=AXIS2_PLACEMENT_3D ( 'NONE', #655, #228, #2462 ) ;
#1684=ADVANCED_FACE ( 'NONE', ( #2450, #2466 ), #220, .T. ) ;
#1690=DIRECTION ( 'NONE',  ( 0.000000000000000000, 0.000000000000000000, 1.000000000000000000 ) ) ;
#1692=VECTOR ( 'NONE', #891, 1000.000000000000000 ) ;
#1698=CARTESIAN_POINT ( 'NONE',  ( 35.00000000000002132, -24.99999999999999645, 3.000000000000011990 ) ) ;
#1699=ORIENTED_EDGE ( 'NONE', *, *, #1201, .F. ) ;
#1704=VERTEX_POINT ( 'NONE', #443 ) ;
#1708=PRODUCT_CONTEXT ( 'NONE', #2613, 'mechanical' ) ;
#1725=FACE_OUTER_BOUND ( 'NONE', #264, .T. ) ;
#1731=FACE_OUTER_BOUND ( 'NONE', #1008, .T. ) ;
#1737=EDGE_LOOP ( 'NONE', ( #41, #1957, #2619, #2781 ) ) ;
#1741=LINE ( 'NONE', #2180, #2704 ) ;
#1743=LINE ( 'NONE', #839, #2523 ) ;
#1747=ORIENTED_EDGE ( 'NONE', *, *, #892, .T. ) ;
#1756=DIRECTION ( 'NONE',  ( 0.000000000000000000, 1.000000000000000000, 0.000000000000000000 ) ) ;
#1757=ORIENTED_EDGE ( 'NONE', *, *, #2016, .T. ) ;
#1763=EDGE_CURVE ( 'NONE', #1101, #2799, #383, .T. ) ;
#1764=ORIENTED_EDGE ( 'NONE', *, *, #1264, .F. ) ;
#1776=DIRECTION ( 'NONE',  ( -0.000000000000000000, -1.000000000000000000, -0.000000000000000000 ) ) ;
#1777=ORIENTED_EDGE ( 'NONE', *, *, #1097, .F. ) ;
#1780=DIRECTION ( 'NONE',  ( -1.000000000000000000, 0.000000000000000000, 0.000000000000000000 ) ) ;
#1784=DIRECTION ( 'NONE',  ( 0.000000000000000000, 0.000000000000000000, 1.000000000000000000 ) ) ;
#1791=EDGE_CURVE ( 'NONE', #1043, #998, #1888, .T. ) ;
#1795=CARTESIAN_POINT ( 'NONE',  ( -39.99999999999999289, -20.00000000000000000, -3.000000000000000000 ) ) ;
#1799=( LENGTH_UNIT ( ) NAMED_UNIT ( * ) SI_UNIT ( .MILLI., .METRE. ) );
#1801=ORIENTED_EDGE ( 'NONE', *, *, #787, .F. ) ;
#1826=DIRECTION ( 'NONE',  ( -2.312964634635742661E-15, 0.000000000000000000, -1.000000000000000000 ) ) ;
#1827=SURFACE_STYLE_USAGE ( .BOTH. , #40 ) ;
#1830=LINE ( 'NONE', #2787, #2381 ) ;
#1841=FACE_OUTER_BOUND ( 'NONE', #661, .T. ) ;
#1844=CIRCLE ( 'NONE', #299, 5.000000000000000000 ) ;
#1846=AXIS2_PLACEMENT_3D ( 'NONE', #1196, #2107, #2077 ) ;
#1847=ORIENTED_EDGE ( 'NONE', *, *, #1097, .T. ) ;
#1848=EDGE_CURVE ( 'NONE', #327, #1043, #292, .T. ) ;
#1851=LINE ( 'NONE', #1878, #1029 ) ;
#1854=EDGE_CURVE ( 'NONE', #937, #1900, #1393, .T. ) ;
#1862=CARTESIAN_POINT ( 'NONE',  ( 35.00000000000001421, -30.00000000000000000, -3.000000000000000000 ) ) ;
#1863=DIRECTION ( 'NONE',  ( 1.000000000000000000, 0.000000000000000000, -0.000000000000000000 ) ) ;
#1877=AXIS2_PLACEMENT_3D ( 'NONE', #498, #1153, #2550 ) ;
#1878=CARTESIAN_POINT ( 'NONE',  ( -39.99999999999999289, -20.00000000000000000, 3.000000000000000000 ) ) ;
#1881=FACE_OUTER_BOUND ( 'NONE', #2603, .T. ) ;
#1887=DIRECTION ( 'NONE',  ( 0.000000000000000000, 1.000000000000000000, 0.000000000000000000 ) ) ;
#1888=CIRCLE ( 'NONE', #2657, 5.000000000000000888 ) ;
#1894=AXIS2_PLACEMENT_3D ( 'NONE', #468, #1618, #2537 ) ;
#1896=DIRECTION ( 'NONE',  ( 0.000000000000000000, 0.000000000000000000, 1.000000000000000000 ) ) ;
#1900=VERTEX_POINT ( 'NONE', #2059 ) ;
#1908=ORIENTED_EDGE ( 'NONE', *, *, #2163, .T. ) ;
#1915=CARTESIAN_POINT ( 'NONE',  ( 35.00000000000001421, -30.00000000000000000, 3.000000000000000000 ) ) ;
#1919=CARTESIAN_POINT ( 'NONE',  ( 0.000000000000000000, -20.00000000000000000, 7.500000000000000888 ) ) ;
#1920=SHAPE_REPRESENTATION_RELATIONSHIP ( 'NONE' , 'NONE' ,  #2004, #1110 ) ;
#1922=AXIS2_PLACEMENT_3D ( 'NONE', #2208, #1756, #2680 ) ;
#1923=CYLINDRICAL_SURFACE ( 'NONE', #2365, 5.000000000000000000 ) ;
#1925=EDGE_CURVE ( 'NONE', #2864, #2373, #328, .T. ) ;
#1935=EDGE_CURVE ( 'NONE', #2373, #237, #1475, .T. ) ;
#1946=DIRECTION ( 'NONE',  ( 1.000000000000000000, 0.000000000000000000, 0.000000000000000000 ) ) ;
#1949=CARTESIAN_POINT ( 'NONE',  ( 35.00000000000002132, -24.99999999999999645, 3.000000000000000000 ) ) ;
#1951=VERTEX_POINT ( 'NONE', #99 ) ;
#1957=ORIENTED_EDGE ( 'NONE', *, *, #2916, .T. ) ;
#1964=EDGE_LOOP ( 'NONE', ( #130, #304, #989, #619 ) ) ;
#1973=AXIS2_PLACEMENT_3D ( 'NONE', #2196, #2618, #822 ) ;
#1976=CARTESIAN_POINT ( 'NONE',  ( 34.00000000000000000, -25.00000000000000000, -3.000000000000000000 ) ) ;
#1984=CARTESIAN_POINT ( 'NONE',  ( 0.000000000000000000, -30.00000000000000000, 0.000000000000000000 ) ) ;
#1989=LINE ( 'NONE', #861, #1692 ) ;
#1991=ORIENTED_EDGE ( 'NONE', *, *, #2594, .F. ) ;
#1993=CARTESIAN_POINT ( 'NONE',  ( 35.00000000000000711, -25.00000000000000000, -3.000000000000000000 ) ) ;
#2003=CARTESIAN_POINT ( 'NONE',  ( 0.000000000000000000, -30.00000000000000000, 0.000000000000000000 ) ) ;
#2004=SHAPE_REPRESENTATION ( 'Central Crosshead Yoke Bar', ( #2652 ), #465 ) ;
#2012=DIRECTION ( 'NONE',  ( -1.000000000000000000, -0.000000000000000000, -0.000000000000000000 ) ) ;
#2014=DIRECTION ( 'NONE',  ( 0.000000000000000000, 1.000000000000000000, 0.000000000000000000 ) ) ;
#2016=EDGE_CURVE ( 'NONE', #2441, #1704, #2377, .T. ) ;
#2028=MECHANICAL_DESIGN_GEOMETRIC_PRESENTATION_REPRESENTATION('',(#97),#285);
#2031=DIRECTION ( 'NONE',  ( 0.000000000000000000, 0.000000000000000000, 1.000000000000000000 ) ) ;
#2032=( GEOMETRIC_REPRESENTATION_CONTEXT ( 3 ) GLOBAL_UNCERTAINTY_ASSIGNED_CONTEXT ( ( #1334 ) ) GLOBAL_UNIT_ASSIGNED_CONTEXT ( ( #778, #2170, #1231 ) ) REPRESENTATION_CONTEXT ( 'NONE', 'WORKASPACE' ) );
#2034=VECTOR ( 'NONE', #1150, 1000.000000000000000 ) ;
#2037=AXIS2_PLACEMENT_3D ( 'NONE', #901, #2271, #2434 ) ;
#2041=EDGE_LOOP ( 'NONE', ( #2551, #64, #407, #275 ) ) ;
#2045=ORIENTED_EDGE ( 'NONE', *, *, #532, .T. ) ;
#2050=ORIENTED_EDGE ( 'NONE', *, *, #1484, .T. ) ;
#2051=UNCERTAINTY_MEASURE_WITH_UNIT (LENGTH_MEASURE( 1.000000000000000082E-05 ), #2879, 'distance_accuracy_value', 'NONE');
#2054=EDGE_LOOP ( 'NONE', ( #2769, #1764 ) ) ;
#2055=FACE_BOUND ( 'NONE', #165, .T. ) ;
#2059=CARTESIAN_POINT ( 'NONE',  ( -39.99999999999999289, -25.00000000000000000, -3.000000000000000000 ) ) ;
#2060=SURFACE_STYLE_FILL_AREA ( #2511 ) ;
#2073=VECTOR ( 'NONE', #323, 1000.000000000000000 ) ;
#2076=CIRCLE ( 'NONE', #1922, 7.500000000000000888 ) ;
#2077=DIRECTION ( 'NONE',  ( 1.000000000000000000, 0.000000000000000000, 0.000000000000000000 ) ) ;
#2082=ORIENTED_EDGE ( 'NONE', *, *, #490, .F. ) ;
#2086=DIRECTION ( 'NONE',  ( 0.000000000000000000, 0.000000000000000000, -1.000000000000000000 ) ) ;
#2091=CARTESIAN_POINT ( 'NONE',  ( -39.99999999999999289, -25.00000000000000000, 3.000000000000000000 ) ) ;
#2093=VERTEX_POINT ( 'NONE', #899 ) ;
#2098=LINE ( 'NONE', #1445, #2073 ) ;
#2099=FACE_OUTER_BOUND ( 'NONE', #929, .T. ) ;
#2101=DIRECTION ( 'NONE',  ( 0.000000000000000000, 0.000000000000000000, -1.000000000000000000 ) ) ;
#2107=DIRECTION ( 'NONE',  ( 0.000000000000000000, 0.000000000000000000, 1.000000000000000000 ) ) ;
#2115=ORIENTED_EDGE ( 'NONE', *, *, #2571, .F. ) ;
#2125=COLOUR_RGB ( '',0.8941176470588234615, 0.8941176470588234615, 0.8941176470588234615 ) ;
#2130=EDGE_CURVE ( 'NONE', #2297, #2864, #2205, .T. ) ;
#2131=LINE ( 'NONE', #2144, #599 ) ;
#2136=AXIS2_PLACEMENT_3D ( 'NONE', #1976, #2689, #1041 ) ;
#2138=VECTOR ( 'NONE', #2349, 1000.000000000000000 ) ;
#2140=ORIENTED_EDGE ( 'NONE', *, *, #1791, .F. ) ;
#2143=ORIENTED_EDGE ( 'NONE', *, *, #738, .F. ) ;
#2144=CARTESIAN_POINT ( 'NONE',  ( 31.35000000000000853, -25.00000000000000000, -3.000000000000000000 ) ) ;
#2149=DIRECTION ( 'NONE',  ( 0.000000000000000000, 0.000000000000000000, 1.000000000000000000 ) ) ;
#2153=EDGE_CURVE ( 'NONE', #1462, #1292, #1643, .T. ) ;
#2163=EDGE_CURVE ( 'NONE', #2668, #772, #1458, .T. ) ;
#2165=DIRECTION ( 'NONE',  ( 1.000000000000000000, 0.000000000000000000, -0.000000000000000000 ) ) ;
#2170=( NAMED_UNIT ( * ) PLANE_ANGLE_UNIT ( ) SI_UNIT ( $, .RADIAN. ) );
#2175=ORIENTED_EDGE ( 'NONE', *, *, #2163, .F. ) ;
#2176=DIRECTION ( 'NONE',  ( 0.000000000000000000, 1.000000000000000000, 0.000000000000000000 ) ) ;
#2180=CARTESIAN_POINT ( 'NONE',  ( 35.00000000000002132, -30.00000000000000000, 3.000000000000011990 ) ) ;
#2181=ORIENTED_EDGE ( 'NONE', *, *, #881, .T. ) ;
#2183=LINE ( 'NONE', #1509, #256 ) ;
#2195=CARTESIAN_POINT ( 'NONE',  ( -39.99999999999999289, -30.00000000000000000, 3.000000000000000000 ) ) ;
#2196=CARTESIAN_POINT ( 'NONE',  ( 34.00000000000000000, -25.00000000000000000, 3.000000000000000000 ) ) ;
#2203=LINE ( 'NONE', #2920, #112 ) ;
#2205=LINE ( 'NONE', #1795, #1302 ) ;
#2207=DIRECTION ( 'NONE',  ( 0.000000000000000000, -0.000000000000000000, 1.000000000000000000 ) ) ;
#2208=CARTESIAN_POINT ( 'NONE',  ( 0.000000000000000000, -30.00000000000000000, 0.000000000000000000 ) ) ;
#2215=CIRCLE ( 'NONE', #644, 5.000000000000000000 ) ;
#2233=VECTOR ( 'NONE', #1346, 1000.000000000000000 ) ;
#2252=ADVANCED_FACE ( 'NONE', ( #50, #940 ), #1390, .F. ) ;
#2266=DIRECTION ( 'NONE',  ( 0.000000000000000000, 0.000000000000000000, -1.000000000000000000 ) ) ;
#2271=DIRECTION ( 'NONE',  ( 0.000000000000000000, 0.000000000000000000, 1.000000000000000000 ) ) ;
#2281=ORIENTED_EDGE ( 'NONE', *, *, #2571, .T. ) ;
#2285=AXIS2_PLACEMENT_3D ( 'NONE', #2669, #209, #1075 ) ;
#2292=PRODUCT_DEFINITION_CONTEXT ( 'detailed design', #1638, 'design' ) ;
#2296=ADVANCED_FACE ( 'NONE', ( #1374, #1841 ), #2779, .T. ) ;
#2297=VERTEX_POINT ( 'NONE', #2748 ) ;
#2304=LINE ( 'NONE', #2806, #2138 ) ;
#2309=CARTESIAN_POINT ( 'NONE',  ( -34.99999999999999289, -20.00000000000000000, 0.000000000000000000 ) ) ;
#2312=AXIS2_PLACEMENT_3D ( 'NONE', #533, #1440, #2347 ) ;
#2321=CARTESIAN_POINT ( 'NONE',  ( -6.873863542433761076, -30.00000000000000000, 3.000000000000000000 ) ) ;
#2341=CARTESIAN_POINT ( 'NONE',  ( 0.000000000000000000, -30.00000000000000000, -5.000000000000000000 ) ) ;
#2343=EDGE_CURVE ( 'NONE', #1558, #772, #2131, .T. ) ;
#2347=DIRECTION ( 'NONE',  ( 0.000000000000000000, 0.000000000000000000, 1.000000000000000000 ) ) ;
#2349=DIRECTION ( 'NONE',  ( -0.000000000000000000, -0.000000000000000000, -1.000000000000000000 ) ) ;
#2352=DIRECTION ( 'NONE',  ( 1.000000000000000000, 0.000000000000000000, 0.000000000000000000 ) ) ;
#2356=VECTOR ( 'NONE', #1378, 1000.000000000000000 ) ;
#2364=DIRECTION ( 'NONE',  ( -0.000000000000000000, -0.000000000000000000, -1.000000000000000000 ) ) ;
#2365=AXIS2_PLACEMENT_3D ( 'NONE', #354, #2827, #1666 ) ;
#2373=VERTEX_POINT ( 'NONE', #1257 ) ;
#2376=DIRECTION ( 'NONE',  ( -1.000000000000000000, 0.000000000000000000, 0.000000000000000000 ) ) ;
#2377=LINE ( 'NONE', #2830, #2838 ) ;
#2378=AXIS2_PLACEMENT_3D ( 'NONE', #451, #2086, #897 ) ;
#2381=VECTOR ( 'NONE', #520, 1000.000000000000000 ) ;
#2382=FACE_OUTER_BOUND ( 'NONE', #115, .T. ) ;
#2383=ADVANCED_FACE ( 'NONE', ( #1203 ), #999, .T. ) ;
#2384=ORIENTED_EDGE ( 'NONE', *, *, #574, .F. ) ;
#2387=EDGE_LOOP ( 'NONE', ( #826, #1215, #1908, #1626 ) ) ;
#2388=ADVANCED_FACE ( 'NONE', ( #1473 ), #1923, .F. ) ;
#2390=CARTESIAN_POINT ( 'NONE',  ( -34.99999999999999289, -25.00000000000000000, -3.000000000000000000 ) ) ;
#2397=CARTESIAN_POINT ( 'NONE',  ( 0.000000000000000000, -19.99999999999999645, -5.000000000000000000 ) ) ;
#2402=ORIENTED_EDGE ( 'NONE', *, *, #1484, .F. ) ;
#2405=VERTEX_POINT ( 'NONE', #2397 ) ;
#2419=CARTESIAN_POINT ( 'NONE',  ( 6.123233995736766282E-16, -19.99999999999999645, 5.000000000000000000 ) ) ;
#2426=ORIENTED_EDGE ( 'NONE', *, *, #2918, .F. ) ;
#2428=EDGE_CURVE ( 'NONE', #2492, #640, #49, .T. ) ;
#2434=DIRECTION ( 'NONE',  ( 1.000000000000000000, 0.000000000000000000, 0.000000000000000000 ) ) ;
#2441=VERTEX_POINT ( 'NONE', #1483 ) ;
#2442=CARTESIAN_POINT ( 'NONE',  ( 0.000000000000000000, -19.99999999999999645, 0.000000000000000000 ) ) ;
#2444=DIRECTION ( 'NONE',  ( 0.000000000000000000, 0.000000000000000000, 1.000000000000000000 ) ) ;
#2450=FACE_BOUND ( 'NONE', #100, .T. ) ;
#2451=ORIENTED_EDGE ( 'NONE', *, *, #293, .T. ) ;
#2458=DIRECTION ( 'NONE',  ( 0.000000000000000000, 0.000000000000000000, -1.000000000000000000 ) ) ;
#2459=ORIENTED_EDGE ( 'NONE', *, *, #246, .T. ) ;
#2462=DIRECTION ( 'NONE',  ( 0.000000000000000000, 0.000000000000000000, -1.000000000000000000 ) ) ;
#2466=FACE_OUTER_BOUND ( 'NONE', #1219, .T. ) ;
#2471=CARTESIAN_POINT ( 'NONE',  ( 31.35000000000001563, -25.00000000000000000, -3.000000000000001332 ) ) ;
#2478=EDGE_LOOP ( 'NONE', ( #2143, #314 ) ) ;
#2488=CARTESIAN_POINT ( 'NONE',  ( 35.00000000000001421, -20.00000000000000000, 3.000000000000000000 ) ) ;
#2492=VERTEX_POINT ( 'NONE', #179 ) ;
#2496=ORIENTED_EDGE ( 'NONE', *, *, #769, .T. ) ;
#2511=FILL_AREA_STYLE ('',( #1145 ) ) ;
#2513=CIRCLE ( 'NONE', #1603, 7.500000000000000888 ) ;
#2520=AXIS2_PLACEMENT_3D ( 'NONE', #227, #922, #1401 ) ;
#2523=VECTOR ( 'NONE', #1295, 1000.000000000000000 ) ;
#2534=MANIFOLD_SOLID_BREP ( 'Fillet1', #2853 ) ;
#2535=ADVANCED_FACE ( 'NONE', ( #1731 ), #395, .F. ) ;
#2537=DIRECTION ( 'NONE',  ( -1.000000000000000000, 0.000000000000000000, 0.000000000000000000 ) ) ;
#2540=CARTESIAN_POINT ( 'NONE',  ( 36.64999999999999858, -25.00000000000000000, 3.000000000000000000 ) ) ;
#2542=ORIENTED_EDGE ( 'NONE', *, *, #796, .T. ) ;
#2545=CARTESIAN_POINT ( 'NONE',  ( -34.00000000000000000, -25.00000000000000000, 3.000000000000000000 ) ) ;
#2547=ORIENTED_EDGE ( 'NONE', *, *, #1615, .T. ) ;
#2549=EDGE_CURVE ( 'NONE', #2297, #1043, #331, .T. ) ;
#2550=DIRECTION ( 'NONE',  ( 0.000000000000000000, -0.000000000000000000, 1.000000000000000000 ) ) ;
#2551=ORIENTED_EDGE ( 'NONE', *, *, #1048, .F. ) ;
#2562=CARTESIAN_POINT ( 'NONE',  ( 0.000000000000000000, -30.00000000000000000, -5.000000000000000000 ) ) ;
#2565=CARTESIAN_POINT ( 'NONE',  ( 0.000000000000000000, -30.00000000000000000, 0.000000000000000000 ) ) ;
#2571=EDGE_CURVE ( 'NONE', #2811, #2405, #2215, .T. ) ;
#2573=AXIS2_PLACEMENT_3D ( 'NONE', #1147, #1208, #1159 ) ;
#2578=LINE ( 'NONE', #2562, #2034 ) ;
#2582=ORIENTED_EDGE ( 'NONE', *, *, #1665, .F. ) ;
#2583=DIRECTION ( 'NONE',  ( 0.000000000000000000, 0.000000000000000000, -1.000000000000000000 ) ) ;
#2588=DIRECTION ( 'NONE',  ( -1.000000000000000000, 0.000000000000000000, 0.000000000000000000 ) ) ;
#2593=LINE ( 'NONE', #345, #525 ) ;
#2594=EDGE_CURVE ( 'NONE', #110, #1556, #1629, .T. ) ;
#2596=AXIS2_PLACEMENT_3D ( 'NONE', #170, #2723, #1780 ) ;
#2603=EDGE_LOOP ( 'NONE', ( #1312, #442, #1404, #174 ) ) ;
#2613=APPLICATION_CONTEXT ( 'automotive_design' ) ;
#2616=CIRCLE ( 'NONE', #1327, 2.649999999999985700 ) ;
#2618=DIRECTION ( 'NONE',  ( 0.000000000000000000, 0.000000000000000000, 1.000000000000000000 ) ) ;
#2619=ORIENTED_EDGE ( 'NONE', *, *, #65, .F. ) ;
#2625=EDGE_CURVE ( 'NONE', #2914, #640, #2098, .T. ) ;
#2627=VERTEX_POINT ( 'NONE', #2321 ) ;
#2629=SHAPE_DEFINITION_REPRESENTATION ( #1184, #2004 ) ;
#2632=DIRECTION ( 'NONE',  ( 1.000000000000000000, 0.000000000000000000, 0.000000000000000000 ) ) ;
#2652=AXIS2_PLACEMENT_3D ( 'NONE', #231, #2031, #1309 ) ;
#2657=AXIS2_PLACEMENT_3D ( 'NONE', #1609, #1655, #276 ) ;
#2659=DIRECTION ( 'NONE',  ( 0.000000000000000000, 0.000000000000000000, 1.000000000000000000 ) ) ;
#2668=VERTEX_POINT ( 'NONE', #297 ) ;
#2669=CARTESIAN_POINT ( 'NONE',  ( 34.00000000000000000, -25.00000000000000000, 3.000000000000000000 ) ) ;
#2675=CARTESIAN_POINT ( 'NONE',  ( -34.99999999999999289, -25.00000000000000000, 3.000000000000000000 ) ) ;
#2680=DIRECTION ( 'NONE',  ( 0.000000000000000000, 0.000000000000000000, 1.000000000000000000 ) ) ;
#2687=DIRECTION ( 'NONE',  ( 0.000000000000000000, 0.000000000000000000, -1.000000000000000000 ) ) ;
#2689=DIRECTION ( 'NONE',  ( -0.000000000000000000, -0.000000000000000000, -1.000000000000000000 ) ) ;
#2697=CARTESIAN_POINT ( 'NONE',  ( -6.873863542433761076, -30.00000000000000000, 3.000000000000000000 ) ) ;
#2703=EDGE_CURVE ( 'NONE', #640, #415, #377, .T. ) ;
#2704=VECTOR ( 'NONE', #573, 1000.000000000000000 ) ;
#2723=DIRECTION ( 'NONE',  ( -0.000000000000000000, -0.000000000000000000, -1.000000000000000000 ) ) ;
#2738=EDGE_LOOP ( 'NONE', ( #450, #2175 ) ) ;
#2739=LINE ( 'NONE', #1612, #1183 ) ;
#2748=CARTESIAN_POINT ( 'NONE',  ( 35.00000000000001421, -20.00000000000000000, -3.000000000000000000 ) ) ;
#2763=CARTESIAN_POINT ( 'NONE',  ( 6.873863542433761076, -20.00000000000000000, 3.000000000000000000 ) ) ;
#2769=ORIENTED_EDGE ( 'NONE', *, *, #1763, .F. ) ;
#2772=DIRECTION ( 'NONE',  ( -0.000000000000000000, -0.000000000000000000, -1.000000000000000000 ) ) ;
#2779=PLANE ( 'NONE',  #461 ) ;
#2781=ORIENTED_EDGE ( 'NONE', *, *, #2703, .F. ) ;
#2787=CARTESIAN_POINT ( 'NONE',  ( -39.99999999999999289, -30.00000000000000000, -3.000000000000000000 ) ) ;
#2788=CARTESIAN_POINT ( 'NONE',  ( 6.123233995736766282E-16, -30.00000000000000000, 5.000000000000000000 ) ) ;
#2789=CARTESIAN_POINT ( 'NONE',  ( 0.000000000000000000, -20.00000000000000000, 0.000000000000000000 ) ) ;
#2791=PRODUCT ( 'Central Crosshead Yoke Bar', 'Central Crosshead Yoke Bar', '', ( #1708 ) ) ;
#2793=ADVANCED_FACE ( 'NONE', ( #2382 ), #1031, .T. ) ;
#2795=DIRECTION ( 'NONE',  ( 0.000000000000000000, 1.000000000000000000, 0.000000000000000000 ) ) ;
#2799=VERTEX_POINT ( 'NONE', #1227 ) ;
#2806=CARTESIAN_POINT ( 'NONE',  ( -36.64999999999999858, -25.00000000000000000, -3.000000000000000000 ) ) ;
#2811=VERTEX_POINT ( 'NONE', #2419 ) ;
#2813=DIRECTION ( 'NONE',  ( 0.000000000000000000, 0.000000000000000000, 1.000000000000000000 ) ) ;
#2815=EDGE_CURVE ( 'NONE', #23, #1558, #648, .T. ) ;
#2826=EDGE_CURVE ( 'NONE', #998, #1556, #1741, .T. ) ;
#2827=DIRECTION ( 'NONE',  ( -0.000000000000000000, -1.000000000000000000, -0.000000000000000000 ) ) ;
#2830=CARTESIAN_POINT ( 'NONE',  ( -34.99999999999999289, -30.00000000000000000, -3.000000000000000000 ) ) ;
#2831=EDGE_LOOP ( 'NONE', ( #2426, #1564 ) ) ;
#2838=VECTOR ( 'NONE', #1026, 1000.000000000000000 ) ;
#2840=AXIS2_PLACEMENT_3D ( 'NONE', #2565, #1887, #2813 ) ;
#2841=CARTESIAN_POINT ( 'NONE',  ( 31.35000000000000853, -25.00000000000000000, 3.000000000000000000 ) ) ;
#2844=ORIENTED_EDGE ( 'NONE', *, *, #1848, .T. ) ;
#2846=DIRECTION ( 'NONE',  ( 1.000000000000000000, 0.000000000000000000, 0.000000000000000000 ) ) ;
#2848=AXIS2_PLACEMENT_3D ( 'NONE', #1631, #1434, #1385 ) ;
#2853=CLOSED_SHELL ( 'NONE', ( #426, #1214, #1299, #449, #2383, #244, #2252, #1684, #2296, #1456, #370, #1578, #2388, #2535, #318, #2793, #562, #271, #1623 ) ) ;
#2864=VERTEX_POINT ( 'NONE', #618 ) ;
#2865=ORIENTED_EDGE ( 'NONE', *, *, #852, .T. ) ;
#2873=DIRECTION ( 'NONE',  ( 0.000000000000000000, 0.000000000000000000, 1.000000000000000000 ) ) ;
#2876=DIRECTION ( 'NONE',  ( -1.000000000000000000, 0.000000000000000000, 0.000000000000000000 ) ) ;
#2878=ORIENTED_EDGE ( 'NONE', *, *, #2130, .F. ) ;
#2879=( LENGTH_UNIT ( ) NAMED_UNIT ( * ) SI_UNIT ( .MILLI., .METRE. ) );
#2880=DIRECTION ( 'NONE',  ( 0.000000000000000000, 1.000000000000000000, 0.000000000000000000 ) ) ;
#2890=CARTESIAN_POINT ( 'NONE',  ( 0.000000000000000000, -19.99999999999999645, 0.000000000000000000 ) ) ;
#2893=ORIENTED_EDGE ( 'NONE', *, *, #881, .F. ) ;
#2896=AXIS2_PLACEMENT_3D ( 'NONE', #765, #1673, #2588 ) ;
#2897=ORIENTED_EDGE ( 'NONE', *, *, #2916, .F. ) ;
#2914=VERTEX_POINT ( 'NONE', #458 ) ;
#2916=EDGE_CURVE ( 'NONE', #2914, #110, #2076, .T. ) ;
#2918=EDGE_CURVE ( 'NONE', #1292, #1462, #512, .T. ) ;
#2920=CARTESIAN_POINT ( 'NONE',  ( 6.873863542433761076, -30.00000000000000000, -3.000000000000000000 ) ) ;
#2925=CARTESIAN_POINT ( 'NONE',  ( 6.123233995736766282E-16, -30.00000000000000000, 5.000000000000000000 ) ) ;
#2943=COLOUR_RGB('Light Blue',0.38,0.62,0.78);
#2944=FILL_AREA_STYLE_COLOUR('',#2943);
#2945=FILL_AREA_STYLE('',(#2944));
#2946=SURFACE_STYLE_FILL_AREA(#2945);
#2947=SURFACE_SIDE_STYLE('',(#2946));
#2948=SURFACE_STYLE_USAGE(.BOTH.,#2947);
#2949=PRESENTATION_STYLE_ASSIGNMENT((#2948));
ENDSEC;
END-ISO-10303-21;
